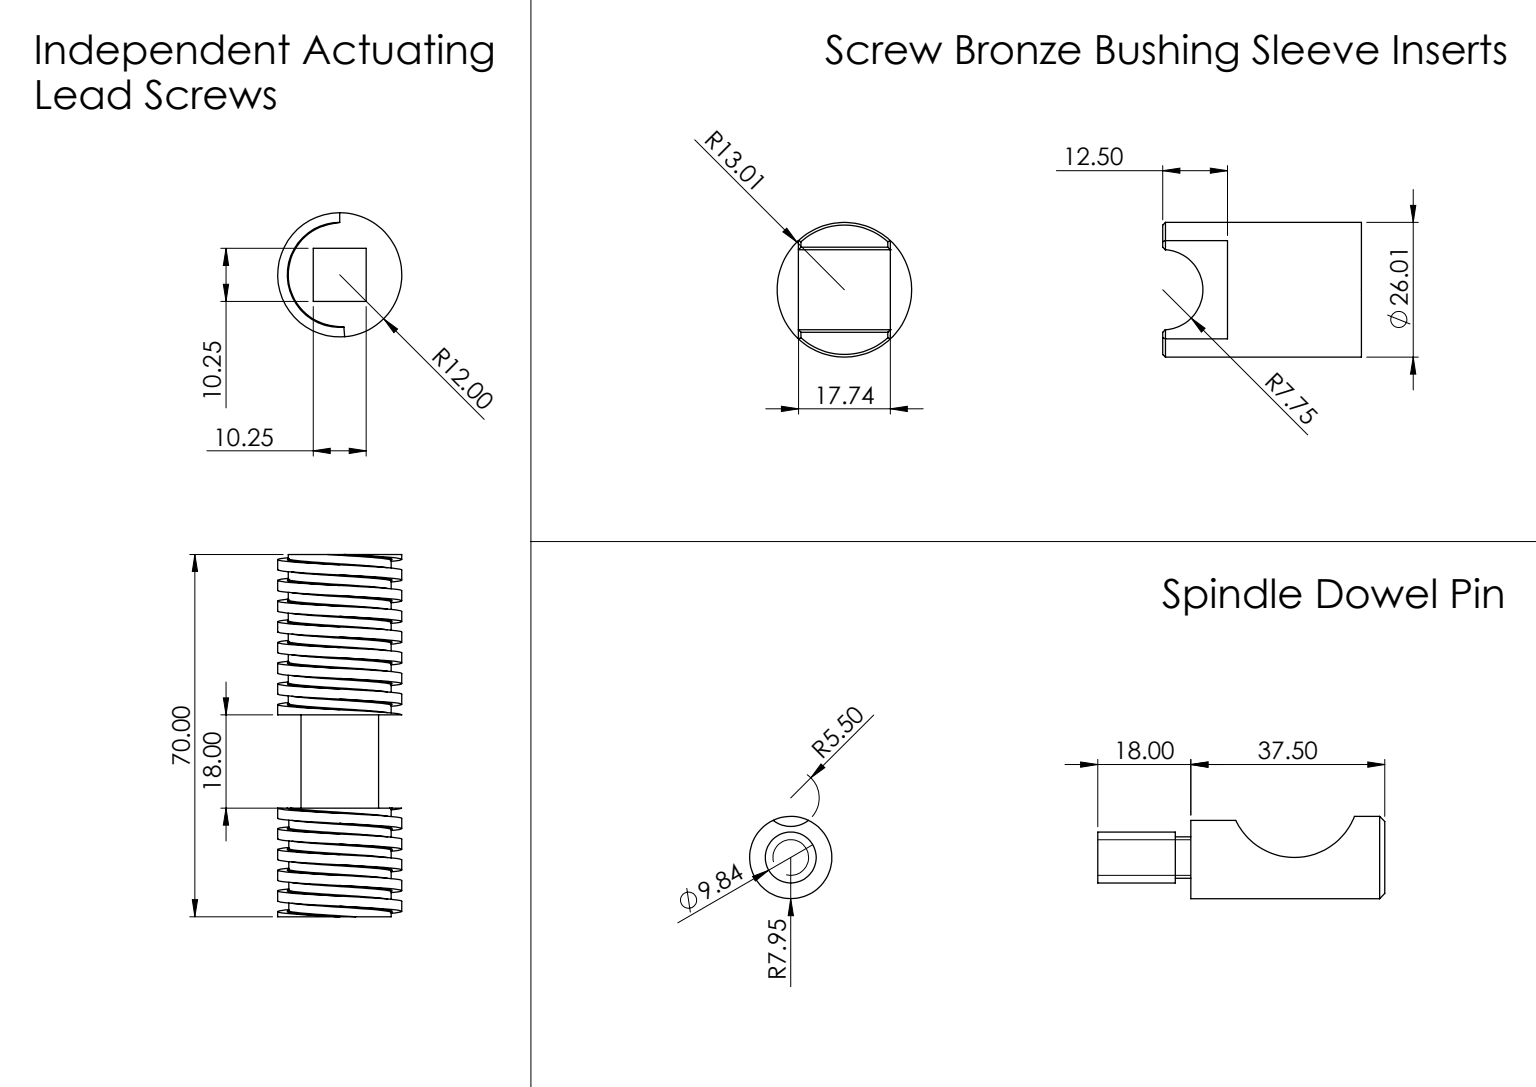
ISO-10303-21;
HEADER;
FILE_DESCRIPTION (('STEP AP214'),
    '1' );
FILE_NAME ('Spindle Dowel Pin.step',
    '2026-10-09T08:48:44',
    ( '' ),
    ( '' ),
    'SwSTEP 2.0',
    'SolidWorks 2026',
    '' );
FILE_SCHEMA (( 'AUTOMOTIVE_DESIGN' ));
ENDSEC;

DATA;
#25=CARTESIAN_POINT ( 'NONE',  ( 2.372150492836604986E-17, 0.000000000000000000, 0.1937007874015747588 ) ) ;
#117=CARTESIAN_POINT ( 'NONE',  ( 0.3074112942705509166, 1.261823755618582510, 0.05913325304464405602 ) ) ;
#225=DIRECTION ( 'NONE',  ( -0.000000000000000000, -1.000000000000000000, -0.000000000000000000 ) ) ;
#301=CARTESIAN_POINT ( 'NONE',  ( 0.000000000000000000, 2.185039370078740273, -0.2736220472440938911 ) ) ;
#383=EDGE_LOOP ( 'NONE', ( #46578, #71434, #76162, #29656 ) ) ;
#409=CARTESIAN_POINT ( 'NONE',  ( 0.01224130022169934474, 1.075705580628688152, 0.2362204724409448231 ) ) ;
#791=DIRECTION ( 'NONE',  ( 0.000000000000000000, 0.000000000000000000, -1.000000000000000000 ) ) ;
#799=DIRECTION ( 'NONE',  ( -0.000000000000000000, -1.000000000000000000, -0.000000000000000000 ) ) ;
#881=AXIS2_PLACEMENT_3D ( 'NONE', #25875, #225, #37687 ) ;
#969=CARTESIAN_POINT ( 'NONE',  ( 0.1341536278048623965, 1.050682278017460725, 0.2827841492639507348 ) ) ;
#1007=CARTESIAN_POINT ( 'NONE',  ( -0.2937696495028822574, 1.187747051217076910, 0.1083477314895111149 ) ) ;
#1152=CARTESIAN_POINT ( 'NONE',  ( 3.591975847892823865E-17, 2.185039370078740273, 0.2736220472440938911 ) ) ;
#1213=ORIENTED_EDGE ( 'NONE', *, *, #76419, .T. ) ;
#1243=VERTEX_POINT ( 'NONE', #14615 ) ;
#1297=ADVANCED_FACE ( 'NONE', ( #26383 ), #52458, .F. ) ;
#1417=CARTESIAN_POINT ( 'NONE',  ( -0.3126853129631109174, 1.368901411070787777, 0.01600703956764241986 ) ) ;
#1453=VERTEX_POINT ( 'NONE', #31866 ) ;
#1534=EDGE_LOOP ( 'NONE', ( #3579, #29369, #48090, #58856 ) ) ;
#2325=STYLED_ITEM ( 'NONE', ( #31329 ), #59000 ) ;
#2374=CARTESIAN_POINT ( 'NONE',  ( 0.3129921259842520787, 1.496062992125984259, 0.000000000000000000 ) ) ;
#2406=DIRECTION ( 'NONE',  ( 0.000000000000000000, 0.000000000000000000, 1.000000000000000000 ) ) ;
#2559=DIRECTION ( 'NONE',  ( 0.000000000000000000, 0.000000000000000000, -1.000000000000000000 ) ) ;
#2625=DIRECTION ( 'NONE',  ( 0.000000000000000000, 1.000000000000000000, 0.000000000000000000 ) ) ;
#2725=CARTESIAN_POINT ( 'NONE',  ( 3.833048050305355326E-17, 1.954428616053095924, 0.3129921259842520787 ) ) ;
#3026=DIRECTION ( 'NONE',  ( 0.000000000000000000, 0.000000000000000000, -1.000000000000000000 ) ) ;
#3140=CARTESIAN_POINT ( 'NONE',  ( 0.3126275856726307700, 1.620602844568471479, 0.01575678725321194573 ) ) ;
#3352=EDGE_CURVE ( 'NONE', #25849, #81942, #50111, .T. ) ;
#3373=VECTOR ( 'NONE', #51517, 39.37007874015748143 ) ;
#3384=FACE_OUTER_BOUND ( 'NONE', #39495, .T. ) ;
#3447=FACE_OUTER_BOUND ( 'NONE', #52967, .T. ) ;
#3556=CARTESIAN_POINT ( 'NONE',  ( 0.07836124490824399047, 1.950604500417927323, 0.3034306265812344305 ) ) ;
#3579=ORIENTED_EDGE ( 'NONE', *, *, #3352, .F. ) ;
#3625=LINE ( 'NONE', #47809, #52958 ) ;
#3671=CYLINDRICAL_SURFACE ( 'NONE', #57254, 0.3129921259842520787 ) ;
#3939=VERTEX_POINT ( 'NONE', #23651 ) ;
#3967=CARTESIAN_POINT ( 'NONE',  ( 0.2909691264735233540, 1.813546053633808830, 0.1157836905918017273 ) ) ;
#4054=CARTESIAN_POINT ( 'NONE',  ( -0.1341536278048670039, 1.050682278017461835, 0.2827841492639485144 ) ) ;
#4079=DIRECTION ( 'NONE',  ( -0.000000000000000000, -1.000000000000000000, -0.000000000000000000 ) ) ;
#4201=CARTESIAN_POINT ( 'NONE',  ( 0.000000000000000000, 2.145669291338582418, -0.3129921259842520787 ) ) ;
#4609=DIRECTION ( 'NONE',  ( 0.000000000000000000, 0.000000000000000000, -1.000000000000000000 ) ) ;
#5256=SURFACE_SIDE_STYLE ('',( #44356 ) ) ;
#5276=CARTESIAN_POINT ( 'NONE',  ( -0.1224964469087656410, 1.944119274041657519, 0.2884380004297487088 ) ) ;
#5295=ORIENTED_EDGE ( 'NONE', *, *, #11474, .F. ) ;
#5671=ORIENTED_EDGE ( 'NONE', *, *, #32566, .T. ) ;
#5679=CARTESIAN_POINT ( 'NONE',  ( 3.833048050305355326E-17, 1.954428616053095924, 0.3129921259842520787 ) ) ;
#5999=AXIS2_PLACEMENT_3D ( 'NONE', #65318, #14396, #38786 ) ;
#6197=ORIENTED_EDGE ( 'NONE', *, *, #68902, .T. ) ;
#6325=AXIS2_PLACEMENT_3D ( 'NONE', #24341, #42454, #56734 ) ;
#6346=ADVANCED_FACE ( 'NONE', ( #36689, #61550 ), #81335, .T. ) ;
#6925=LINE ( 'NONE', #78486, #3373 ) ;
#7227=ORIENTED_EDGE ( 'NONE', *, *, #28583, .T. ) ;
#7263=CARTESIAN_POINT ( 'NONE',  ( 0.3104096989839266740, 1.295945406154406454, 0.04180176832660051356 ) ) ;
#7469=DIRECTION ( 'NONE',  ( -0.000000000000000000, -1.000000000000000000, -0.000000000000000000 ) ) ;
#7519=VERTEX_POINT ( 'NONE', #4201 ) ;
#7675=VECTOR ( 'NONE', #22908, 39.37007874015748143 ) ;
#7733=CARTESIAN_POINT ( 'NONE',  ( -0.3129921259842520231, 1.470107679032609971, 3.734948428837856094E-17 ) ) ;
#7767=CARTESIAN_POINT ( 'NONE',  ( 0.000000000000000000, 0.000000000000000000, 0.000000000000000000 ) ) ;
#7885=ORIENTED_EDGE ( 'NONE', *, *, #20353, .F. ) ;
#7890=CARTESIAN_POINT ( 'NONE',  ( -0.04868480690927201593, 1.072582076400621753, 0.2414116071904397476 ) ) ;
#7943=ADVANCED_FACE ( 'NONE', ( #3384 ), #56554, .T. ) ;
#8076=ORIENTED_EDGE ( 'NONE', *, *, #32566, .F. ) ;
#8107=CARTESIAN_POINT ( 'NONE',  ( 0.2748794045270251951, 1.142111962221293409, 0.1499919135227574252 ) ) ;
#8145=CARTESIAN_POINT ( 'NONE',  ( -0.2835710216259798577, 1.159555538018685716, 0.1328243903749163624 ) ) ;
#8310=DIRECTION ( 'NONE',  ( 1.000000000000000000, -0.000000000000000000, -0.000000000000000000 ) ) ;
#8366=PRODUCT ( 'Spindle Dowel Pin', 'Spindle Dowel Pin', '', ( #30024 ) ) ;
#8391=CARTESIAN_POINT ( 'NONE',  ( 0.1341536278048623965, 1.050682278017460725, 0.2827841492639507348 ) ) ;
#8564=ORIENTED_EDGE ( 'NONE', *, *, #32130, .F. ) ;
#8617=VERTEX_POINT ( 'NONE', #32503 ) ;
#8933=PLANE ( 'NONE',  #11755 ) ;
#8939=CIRCLE ( 'NONE', #74851, 0.1937007874015748143 ) ;
#8988=EDGE_CURVE ( 'NONE', #3939, #18816, #67404, .T. ) ;
#9096=EDGE_LOOP ( 'NONE', ( #28412, #46874, #14400, #76473, #66041, #66129, #8076 ) ) ;
#9136=CARTESIAN_POINT ( 'NONE',  ( 0.000000000000000000, 0.000000000000000000, 0.000000000000000000 ) ) ;
#9758=AXIS2_PLACEMENT_3D ( 'NONE', #68690, #23649, #53976 ) ;
#9868=CARTESIAN_POINT ( 'NONE',  ( 0.3130345246323552599, 1.559122693537392745, 0.003049358274158167365 ) ) ;
#10309=ADVANCED_FACE ( 'NONE', ( #27240 ), #73542, .F. ) ;
#10351=SURFACE_STYLE_USAGE ( .BOTH. , #5256 ) ;
#10361=EDGE_LOOP ( 'NONE', ( #73166, #30222 ) ) ;
#10364=DIRECTION ( 'NONE',  ( 0.000000000000000000, 0.000000000000000000, -1.000000000000000000 ) ) ;
#10589=DIRECTION ( 'NONE',  ( 0.000000000000000000, -1.000000000000000000, 0.000000000000000000 ) ) ;
#10777=CARTESIAN_POINT ( 'NONE',  ( -0.3072632741606444173, 1.737537999042348513, 0.06216925787398272507 ) ) ;
#11014=ADVANCED_FACE ( 'NONE', ( #38097 ), #76103, .T. ) ;
#11188=CARTESIAN_POINT ( 'NONE',  ( 0.000000000000000000, 0.5905511811023621549, -0.1937007874015747588 ) ) ;
#11190=CARTESIAN_POINT ( 'NONE',  ( -0.2493074132419488831, 1.884549279140503408, 0.1897364805620621597 ) ) ;
#11276=ORIENTED_EDGE ( 'NONE', *, *, #37551, .F. ) ;
#11474=EDGE_CURVE ( 'NONE', #16433, #18816, #43794, .T. ) ;
#11755=AXIS2_PLACEMENT_3D ( 'NONE', #72906, #2625, #79656 ) ;
#11869=CIRCLE ( 'NONE', #50650, 0.3129921259842521897 ) ;
#12372=ADVANCED_FACE ( 'NONE', ( #28796 ), #80173, .F. ) ;
#12411=EDGE_LOOP ( 'NONE', ( #77639, #27414 ) ) ;
#12421=CARTESIAN_POINT ( 'NONE',  ( -0.1887375355206090954, 1.924695534443318090, 0.2501427588384230183 ) ) ;
#12546=AXIS2_PLACEMENT_3D ( 'NONE', #74485, #47545, #54688 ) ;
#12711=EDGE_LOOP ( 'NONE', ( #79365, #14090, #71316, #31641, #37257 ) ) ;
#13043=CARTESIAN_POINT ( 'NONE',  ( 0.02439311036560904908, 1.075073066373593234, 0.2372510453448407330 ) ) ;
#13195=CARTESIAN_POINT ( 'NONE',  ( 0.1341536278048623410, 0.7086614173228346081, 0.2827841492639508458 ) ) ;
#13216=CARTESIAN_POINT ( 'NONE',  ( -0.3130110660353679908, 1.444485302887537514, 0.002040369744756952066 ) ) ;
#13353=CARTESIAN_POINT ( 'NONE',  ( 0.000000000000000000, 0.5905511811023621549, 0.000000000000000000 ) ) ;
#13876=DIRECTION ( 'NONE',  ( 0.000000000000000000, -0.7071067811865437980, -0.7071067811865511255 ) ) ;
#14020=CIRCLE ( 'NONE', #24744, 0.1574803149606299746 ) ;
#14090=ORIENTED_EDGE ( 'NONE', *, *, #52104, .T. ) ;
#14206=VERTEX_POINT ( 'NONE', #68041 ) ;
#14207=EDGE_LOOP ( 'NONE', ( #60952, #75599, #55224, #46243, #18435, #5295, #68335 ) ) ;
#14304=CARTESIAN_POINT ( 'NONE',  ( -2.199130528046420221E-22, 1.075705580628688596, 0.2362204724409449064 ) ) ;
#14378=VERTEX_POINT ( 'NONE', #4054 ) ;
#14396=DIRECTION ( 'NONE',  ( 1.000000000000000000, -0.000000000000000000, -0.000000000000000000 ) ) ;
#14400=ORIENTED_EDGE ( 'NONE', *, *, #56918, .T. ) ;
#14472=CARTESIAN_POINT ( 'NONE',  ( -0.3064070226227782467, 1.250422264350145474, 0.06492945659560576954 ) ) ;
#14549=EDGE_CURVE ( 'NONE', #39843, #58335, #44637, .T. ) ;
#14607=DIRECTION ( 'NONE',  ( -0.000000000000000000, -1.000000000000000000, -0.000000000000000000 ) ) ;
#14615=CARTESIAN_POINT ( 'NONE',  ( 3.833048052449394218E-17, 2.145669291338582418, 0.3129921259842520787 ) ) ;
#14719=CARTESIAN_POINT ( 'NONE',  ( 0.09404056145105300912, 1.063503333403748474, 0.2573448916946036724 ) ) ;
#14869=ADVANCED_FACE ( 'NONE', ( #3447 ), #8933, .T. ) ;
#15024=LINE ( 'NONE', #40680, #28369 ) ;
#15036=CARTESIAN_POINT ( 'NONE',  ( -0.06038700950485487162, 1.070773487107445909, 0.2444607762650621019 ) ) ;
#15218=VERTEX_POINT ( 'NONE', #71137 ) ;
#15385=EDGE_LOOP ( 'NONE', ( #22971, #11276 ) ) ;
#15414=VERTEX_POINT ( 'NONE', #64400 ) ;
#15463=DIRECTION ( 'NONE',  ( 0.000000000000000000, 0.000000000000000000, -1.000000000000000000 ) ) ;
#15486=CARTESIAN_POINT ( 'NONE',  ( 0.000000000000000000, -1.268531780058464091E-17, 0.000000000000000000 ) ) ;
#15994=B_SPLINE_CURVE_WITH_KNOTS ( 'NONE', 3,
 ( #8391, #26493, #78693, #14719, #77427, #52563, #51725, #13043, #409, #14304 ),
 .UNSPECIFIED., .F., .F.,
 ( 4, 2, 2, 2, 4 ),
 ( 0.001464733143057391418, 0.002397049282983275756, 0.003329365422909159877, 0.004261681562835043131, 0.005193997702760927253 ),
 .UNSPECIFIED. ) ;
#16286=SHAPE_REPRESENTATION_RELATIONSHIP ( 'NONE' , 'NONE' ,  #76132, #64521 ) ;
#16312=DIRECTION ( 'NONE',  ( 0.000000000000000000, 0.000000000000000000, -1.000000000000000000 ) ) ;
#16433=VERTEX_POINT ( 'NONE', #55908 ) ;
#16485=EDGE_CURVE ( 'NONE', #1243, #7519, #53371, .T. ) ;
#16560=CARTESIAN_POINT ( 'NONE',  ( -0.1341536278048623410, 0.7086614173228346081, 0.2827841492639507903 ) ) ;
#16609=CARTESIAN_POINT ( 'NONE',  ( 0.2009426810023753340, 1.919101783098011715, 0.2404105009256824188 ) ) ;
#16873=DIRECTION ( 'NONE',  ( -0.000000000000000000, -1.000000000000000000, -0.000000000000000000 ) ) ;
#17028=CARTESIAN_POINT ( 'NONE',  ( 0.2320225394537987207, 1.899862155193571711, 0.2105147107788077343 ) ) ;
#17085=FILL_AREA_STYLE ('',( #74737 ) ) ;
#17106=CARTESIAN_POINT ( 'NONE',  ( -0.2867050620510094849, 1.825346416092846091, 0.1260848743807634342 ) ) ;
#17210=PLANE ( 'NONE',  #57386 ) ;
#17274=DIRECTION ( 'NONE',  ( -0.000000000000000000, -1.000000000000000000, -0.000000000000000000 ) ) ;
#17515=CARTESIAN_POINT ( 'NONE',  ( -0.2570577095524356759, 1.875999552332453746, 0.1790154821377908934 ) ) ;
#17897=EDGE_CURVE ( 'NONE', #75063, #3939, #42675, .T. ) ;
#17903=( NAMED_UNIT ( * ) SI_UNIT ( $, .STERADIAN. ) SOLID_ANGLE_UNIT ( ) );
#17914=ORIENTED_EDGE ( 'NONE', *, *, #3352, .T. ) ;
#17922=CARTESIAN_POINT ( 'NONE',  ( -0.3129921259842520787, 1.496062992125984259, 2.300774849103979725E-17 ) ) ;
#18007=ORIENTED_EDGE ( 'NONE', *, *, #11474, .T. ) ;
#18252=CARTESIAN_POINT ( 'NONE',  ( 0.000000000000000000, 0.000000000000000000, 0.000000000000000000 ) ) ;
#18429=DIRECTION ( 'NONE',  ( 0.000000000000000000, 0.000000000000000000, -1.000000000000000000 ) ) ;
#18435=ORIENTED_EDGE ( 'NONE', *, *, #32130, .T. ) ;
#18636=DIRECTION ( 'NONE',  ( 0.000000000000000000, 1.000000000000000000, 0.000000000000000000 ) ) ;
#18816=VERTEX_POINT ( 'NONE', #13195 ) ;
#19735=ORIENTED_EDGE ( 'NONE', *, *, #20396, .F. ) ;
#19797=AXIS2_PLACEMENT_3D ( 'NONE', #23157, #16873, #61876 ) ;
#19980=EDGE_CURVE ( 'NONE', #39843, #75063, #15994, .T. ) ;
#20353=EDGE_CURVE ( 'NONE', #49008, #14378, #70690, .T. ) ;
#20385=DIRECTION ( 'NONE',  ( 0.000000000000000000, 0.000000000000000000, -1.000000000000000000 ) ) ;
#20396=EDGE_CURVE ( 'NONE', #31638, #7519, #45830, .T. ) ;
#20602=CARTESIAN_POINT ( 'NONE',  ( 0.000000000000000000, 0.000000000000000000, 0.000000000000000000 ) ) ;
#20680=ORIENTED_EDGE ( 'NONE', *, *, #53659, .T. ) ;
#20733=CARTESIAN_POINT ( 'NONE',  ( 0.2527386706991758825, 1.111414106920971090, 0.1849575905693944811 ) ) ;
#20828=DIRECTION ( 'NONE',  ( 0.000000000000000000, 0.000000000000000000, -1.000000000000000000 ) ) ;
#21132=COLOUR_RGB ( '', 0.08235294, 0.09019608, 0.10196078) ;
#21148=CARTESIAN_POINT ( 'NONE',  ( 0.3114547874990893916, 1.319604222443112151, 0.03199850469859417956 ) ) ;
#21435=VERTEX_POINT ( 'NONE', #11188 ) ;
#21647=DIRECTION ( 'NONE',  ( 0.000000000000000000, 0.000000000000000000, -1.000000000000000000 ) ) ;
#21660=CARTESIAN_POINT ( 'NONE',  ( 0.2979138814448422101, 1.789193252437325743, 0.09652054087235428792 ) ) ;
#21737=DIRECTION ( 'NONE',  ( -0.000000000000000000, -1.000000000000000000, -0.000000000000000000 ) ) ;
#21748=CARTESIAN_POINT ( 'NONE',  ( -0.02462164107398554652, 1.075056246094946211, 0.2372787660107268937 ) ) ;
#21844=CARTESIAN_POINT ( 'NONE',  ( 0.1341536278048623965, 1.050682278017460725, 0.2827841492639507348 ) ) ;
#22077=CARTESIAN_POINT ( 'NONE',  ( 0.1230917936933036416, 1.944006284485450209, 0.2881873359806741419 ) ) ;
#22098=AXIS2_PLACEMENT_3D ( 'NONE', #9136, #2406, #28064 ) ;
#22901=CARTESIAN_POINT ( 'NONE',  ( 0.3095674345919382509, 1.709700804348449843, 0.04767548262574627937 ) ) ;
#22908=DIRECTION ( 'NONE',  ( -0.000000000000000000, -1.000000000000000000, -0.000000000000000000 ) ) ;
#22971=ORIENTED_EDGE ( 'NONE', *, *, #57708, .F. ) ;
#23157=CARTESIAN_POINT ( 'NONE',  ( 0.000000000000000000, 0.000000000000000000, 0.000000000000000000 ) ) ;
#23169=ORIENTED_EDGE ( 'NONE', *, *, #28151, .T. ) ;
#23314=CARTESIAN_POINT ( 'NONE',  ( 0.2451238321738833381, 1.888229281464673948, 0.1947436408813261743 ) ) ;
#23327=DIRECTION ( 'NONE',  ( 8.659560562354975999E-17, -0.7071067811865437980, 0.7071067811865511255 ) ) ;
#23385=FACE_OUTER_BOUND ( 'NONE', #1534, .T. ) ;
#23649=DIRECTION ( 'NONE',  ( 0.000000000000000000, -1.000000000000000000, -0.000000000000000000 ) ) ;
#23651=CARTESIAN_POINT ( 'NONE',  ( 0.000000000000000000, 0.7086614173228346081, 0.2362204724409449064 ) ) ;
#23816=( CONVERSION_BASED_UNIT ( 'INCH', #36040 ) LENGTH_UNIT ( ) NAMED_UNIT ( #43771 ) );
#23849=CARTESIAN_POINT ( 'NONE',  ( 1.928577636452524918E-17, 0.000000000000000000, 0.1574803149606299746 ) ) ;
#24212=CARTESIAN_POINT ( 'NONE',  ( -0.3130349471939997685, 1.559138852304699174, 0.003046472099445048272 ) ) ;
#24317=CARTESIAN_POINT ( 'NONE',  ( 0.1937007874015748143, -6.342658900292320455E-18, 0.000000000000000000 ) ) ;
#24339=AXIS2_PLACEMENT_3D ( 'NONE', #76558, #32762, #791 ) ;
#24341=CARTESIAN_POINT ( 'NONE',  ( 0.000000000000000000, 2.145669291338582418, 0.000000000000000000 ) ) ;
#24430=DIMENSIONAL_EXPONENTS ( 1.000000000000000000, 0.000000000000000000, 0.000000000000000000, 0.000000000000000000, 0.000000000000000000, 0.000000000000000000, 0.000000000000000000 ) ;
#24744=AXIS2_PLACEMENT_3D ( 'NONE', #44138, #17274, #4609 ) ;
#25004=AXIS2_PLACEMENT_3D ( 'NONE', #18252, #31274, #56939 ) ;
#25084=EDGE_CURVE ( 'NONE', #69331, #81942, #62659, .T. ) ;
#25849=VERTEX_POINT ( 'NONE', #81088 ) ;
#25875=CARTESIAN_POINT ( 'NONE',  ( 0.000000000000000000, 2.145669291338582418, 0.000000000000000000 ) ) ;
#25958=DIRECTION ( 'NONE',  ( -0.000000000000000000, -1.000000000000000000, -0.000000000000000000 ) ) ;
#26140=ORIENTED_EDGE ( 'NONE', *, *, #37551, .T. ) ;
#26383=FACE_OUTER_BOUND ( 'NONE', #33205, .T. ) ;
#26401=AXIS2_PLACEMENT_3D ( 'NONE', #40701, #8310, #15463 ) ;
#26492=CYLINDRICAL_SURFACE ( 'NONE', #73490, 0.1937007874015747588 ) ;
#26493=CARTESIAN_POINT ( 'NONE',  ( 0.1249024489578631214, 1.054114278624317835, 0.2754824702603712039 ) ) ;
#26623=CARTESIAN_POINT ( 'NONE',  ( 0.1876687465225647666, 1.067092265285233266, 0.2507773264951494996 ) ) ;
#26693=CYLINDRICAL_SURFACE ( 'NONE', #77547, 0.1574803149606299746 ) ;
#26815=CARTESIAN_POINT ( 'NONE',  ( -0.08317555404016972742, 1.066210426301412717, 0.2524679153701900325 ) ) ;
#27002=ADVANCED_FACE ( 'NONE', ( #66053 ), #26492, .T. ) ;
#27032=CARTESIAN_POINT ( 'NONE',  ( 0.3129921259842522452, 1.470238543415450350, 1.333910153156375395E-19 ) ) ;
#27056=DIRECTION ( 'NONE',  ( 0.000000000000000000, 0.000000000000000000, -1.000000000000000000 ) ) ;
#27240=FACE_OUTER_BOUND ( 'NONE', #12711, .T. ) ;
#27414=ORIENTED_EDGE ( 'NONE', *, *, #49189, .F. ) ;
#27449=CARTESIAN_POINT ( 'NONE',  ( 0.3011055150036106021, 1.218137231435314272, 0.08579257120109930190 ) ) ;
#27907=CARTESIAN_POINT ( 'NONE',  ( -0.3104009647183427756, 1.295819047631763254, 0.04186094777090585556 ) ) ;
#28064=DIRECTION ( 'NONE',  ( 1.000000000000000000, 0.000000000000000000, 0.000000000000000000 ) ) ;
#28151=EDGE_CURVE ( 'NONE', #21435, #25849, #45776, .T. ) ;
#28319=CARTESIAN_POINT ( 'NONE',  ( -0.1341536278048670039, 1.050682278017461835, 0.2827841492639485144 ) ) ;
#28369=VECTOR ( 'NONE', #21737, 39.37007874015748143 ) ;
#28412=ORIENTED_EDGE ( 'NONE', *, *, #36496, .F. ) ;
#28496=UNCERTAINTY_MEASURE_WITH_UNIT (LENGTH_MEASURE( 1.000000000000000082E-05 ), #81468, 'distance_accuracy_value', 'NONE');
#28541=VERTEX_POINT ( 'NONE', #1152 ) ;
#28583=EDGE_CURVE ( 'NONE', #1453, #8617, #30996, .T. ) ;
#28796=FACE_OUTER_BOUND ( 'NONE', #68835, .T. ) ;
#28803=CARTESIAN_POINT ( 'NONE',  ( 0.2570685524539542688, 1.875513320822418839, 0.1786727789893264307 ) ) ;
#28886=PRODUCT_DEFINITION_FORMATION_WITH_SPECIFIED_SOURCE ( 'ANY', '', #8366, .NOT_KNOWN. ) ;
#28893=FACE_OUTER_BOUND ( 'NONE', #12411, .T. ) ;
#29148=CARTESIAN_POINT ( 'NONE',  ( -0.2589415859896363470, 1.118607810292596705, 0.1761306047597130386 ) ) ;
#29369=ORIENTED_EDGE ( 'NONE', *, *, #49189, .T. ) ;
#29615=SHAPE_DEFINITION_REPRESENTATION ( #60807, #76132 ) ;
#29630=CARTESIAN_POINT ( 'NONE',  ( 0.1083363854164813983, 1.946602136093918745, 0.2940643763633090102 ) ) ;
#29656=ORIENTED_EDGE ( 'NONE', *, *, #53659, .F. ) ;
#30024=PRODUCT_CONTEXT ( 'NONE', #61604, 'mechanical' ) ;
#30068=EDGE_CURVE ( 'NONE', #49008, #3939, #66058, .T. ) ;
#30099=( LENGTH_UNIT ( ) NAMED_UNIT ( * ) SI_UNIT ( $, .METRE. ) );
#30118=CARTESIAN_POINT ( 'NONE',  ( -0.06257671775081299903, 1.952079521258549777, 0.3070762858441002940 ) ) ;
#30222=ORIENTED_EDGE ( 'NONE', *, *, #73238, .T. ) ;
#30517=( NAMED_UNIT ( * ) PLANE_ANGLE_UNIT ( ) SI_UNIT ( $, .RADIAN. ) );
#30555=EDGE_LOOP ( 'NONE', ( #23169, #17914, #39523, #35275 ) ) ;
#30641=FACE_OUTER_BOUND ( 'NONE', #10361, .T. ) ;
#30939=CARTESIAN_POINT ( 'NONE',  ( -0.1637150164629772586, 1.933882213591592736, 0.2671902889294776595 ) ) ;
#30996=CIRCLE ( 'NONE', #80787, 0.1574803149606299746 ) ;
#31274=DIRECTION ( 'NONE',  ( -0.000000000000000000, -1.000000000000000000, -0.000000000000000000 ) ) ;
#31329=PRESENTATION_STYLE_ASSIGNMENT (( #10351 ) ) ;
#31638=VERTEX_POINT ( 'NONE', #301 ) ;
#31641=ORIENTED_EDGE ( 'NONE', *, *, #19980, .F. ) ;
#31866=CARTESIAN_POINT ( 'NONE',  ( 0.000000000000000000, 0.5905511811023621549, -0.1574803149606299746 ) ) ;
#32108=PRODUCT_DEFINITION ( 'UNKNOWN', '', #28886, #61306 ) ;
#32130=EDGE_CURVE ( 'NONE', #39843, #18816, #15024, .T. ) ;
#32293=DIRECTION ( 'NONE',  ( 0.000000000000000000, 0.000000000000000000, -1.000000000000000000 ) ) ;
#32503=CARTESIAN_POINT ( 'NONE',  ( 1.928577636452524918E-17, 0.5905511811023621549, 0.1574803149606299746 ) ) ;
#32511=CARTESIAN_POINT ( 'NONE',  ( 0.2063662664111909073, 1.075973491904217871, 0.2356306219338031305 ) ) ;
#32566=EDGE_CURVE ( 'NONE', #14206, #15218, #40961, .T. ) ;
#32698=DIRECTION ( 'NONE',  ( -0.000000000000000000, -1.000000000000000000, -0.000000000000000000 ) ) ;
#32762=DIRECTION ( 'NONE',  ( 0.000000000000000000, -1.000000000000000000, 0.000000000000000000 ) ) ;
#32895=FACE_OUTER_BOUND ( 'NONE', #54214, .T. ) ;
#32971=CARTESIAN_POINT ( 'NONE',  ( -0.3129921259842520787, 1.496062992125984259, 2.300774849103979725E-17 ) ) ;
#33200=( GEOMETRIC_REPRESENTATION_CONTEXT ( 3 ) GLOBAL_UNCERTAINTY_ASSIGNED_CONTEXT ( ( #28496 ) ) GLOBAL_UNIT_ASSIGNED_CONTEXT ( ( #81468, #30517, #17903 ) ) REPRESENTATION_CONTEXT ( 'NONE', 'WORKASPACE' ) );
#33205=EDGE_LOOP ( 'NONE', ( #48733, #76091, #39632, #8564 ) ) ;
#33330=ORIENTED_EDGE ( 'NONE', *, *, #43286, .T. ) ;
#33362=CARTESIAN_POINT ( 'NONE',  ( 0.2314737228097724919, 1.092014648053644565, 0.2109979669470876118 ) ) ;
#33400=CARTESIAN_POINT ( 'NONE',  ( -0.3128565372736722416, 1.393882159635214890, 0.01004378685656346325 ) ) ;
#33733=EDGE_CURVE ( 'NONE', #31638, #28541, #36477, .T. ) ;
#33773=CARTESIAN_POINT ( 'NONE',  ( 0.3130111271098954262, 1.444537301488023839, 0.002033853763896861528 ) ) ;
#33784=DIRECTION ( 'NONE',  ( -0.000000000000000000, -1.000000000000000000, -0.000000000000000000 ) ) ;
#34267=ORIENTED_EDGE ( 'NONE', *, *, #30068, .T. ) ;
#34422=B_SPLINE_CURVE_WITH_KNOTS ( 'NONE', 3,
 ( #78181, #45743, #21748, #7890, #15036, #26815, #39443, #72688, #46995, #53721 ),
 .UNSPECIFIED., .F., .F.,
 ( 4, 2, 2, 2, 4 ),
 ( 0.005193997702760927253, 0.006123015815168760499, 0.007052033927576592878, 0.007981052039984426125, 0.008910070152392259371 ),
 .UNSPECIFIED. ) ;
#34543=CARTESIAN_POINT ( 'NONE',  ( 0.000000000000000000, 2.145669291338582418, 0.000000000000000000 ) ) ;
#34588=VECTOR ( 'NONE', #37121, 39.37007874015748143 ) ;
#34716=CARTESIAN_POINT ( 'NONE',  ( 0.3129921259842522452, 1.527841585044882100, -3.001297844601851921E-19 ) ) ;
#34834=DIRECTION ( 'NONE',  ( -0.000000000000000000, -1.000000000000000000, -0.000000000000000000 ) ) ;
#35275=ORIENTED_EDGE ( 'NONE', *, *, #79779, .F. ) ;
#35369=DIRECTION ( 'NONE',  ( -0.000000000000000000, -1.000000000000000000, -0.000000000000000000 ) ) ;
#35498=VECTOR ( 'NONE', #4079, 39.37007874015748143 ) ;
#35512=DIRECTION ( 'NONE',  ( 0.000000000000000000, 0.000000000000000000, -1.000000000000000000 ) ) ;
#35515=CIRCLE ( 'NONE', #73132, 0.3129921259842520787 ) ;
#35537=CARTESIAN_POINT ( 'NONE',  ( 0.2868249070713367876, 1.825030329442032917, 0.1258042619966805165 ) ) ;
#35564=EDGE_CURVE ( 'NONE', #58335, #14206, #68976, .T. ) ;
#35627=( LENGTH_UNIT ( ) NAMED_UNIT ( * ) SI_UNIT ( $, .METRE. ) );
#35720=DIRECTION ( 'NONE',  ( 0.000000000000000000, 0.000000000000000000, 1.000000000000000000 ) ) ;
#35884=CARTESIAN_POINT ( 'NONE',  ( -0.1775461242611900137, 1.063099670987233569, 0.2580608039878784510 ) ) ;
#35963=CARTESIAN_POINT ( 'NONE',  ( 0.000000000000000000, 2.185078740157480937, 0.2362204724409449064 ) ) ;
#36040=LENGTH_MEASURE_WITH_UNIT ( LENGTH_MEASURE( 0.02539999999999999897 ), #35627 );
#36127=ORIENTED_EDGE ( 'NONE', *, *, #65474, .T. ) ;
#36288=CARTESIAN_POINT ( 'NONE',  ( -0.2526890999533557003, 1.111360978596734883, 0.1850246388144368703 ) ) ;
#36321=ADVANCED_FACE ( 'NONE', ( #49806 ), #49398, .T. ) ;
#36477=CIRCLE ( 'NONE', #62017, 0.2736220472440938911 ) ;
#36496=EDGE_CURVE ( 'NONE', #1243, #14206, #64935, .T. ) ;
#36689=FACE_OUTER_BOUND ( 'NONE', #65322, .T. ) ;
#36704=LINE ( 'NONE', #62378, #34588 ) ;
#36831=LENGTH_MEASURE_WITH_UNIT ( LENGTH_MEASURE( 0.02539999999999999897 ), #30099 );
#37121=DIRECTION ( 'NONE',  ( 1.000000000000000000, -0.000000000000000000, -0.000000000000000000 ) ) ;
#37257=ORIENTED_EDGE ( 'NONE', *, *, #14549, .T. ) ;
#37260=CYLINDRICAL_SURFACE ( 'NONE', #69081, 0.1937007874015747588 ) ;
#37551=EDGE_CURVE ( 'NONE', #75751, #15414, #39876, .T. ) ;
#37666=CARTESIAN_POINT ( 'NONE',  ( -0.2217488924428978880, 1.907169838053261124, 0.2213636967189943072 ) ) ;
#37687=DIRECTION ( 'NONE',  ( 0.000000000000000000, 0.000000000000000000, -1.000000000000000000 ) ) ;
#38097=FACE_OUTER_BOUND ( 'NONE', #79100, .T. ) ;
#38247=CARTESIAN_POINT ( 'NONE',  ( 0.000000000000000000, 0.000000000000000000, -0.1574803149606299746 ) ) ;
#38252=VECTOR ( 'NONE', #799, 39.37007874015748143 ) ;
#38696=CARTESIAN_POINT ( 'NONE',  ( -0.1341536278048623410, 1.446850393700787274, 0.2827841492639507903 ) ) ;
#38786=DIRECTION ( 'NONE',  ( 0.000000000000000000, 0.000000000000000000, -1.000000000000000000 ) ) ;
#38862=CARTESIAN_POINT ( 'NONE',  ( -0.3034767870060118278, 1.228735513192457551, 0.07815720285223907993 ) ) ;
#39241=CARTESIAN_POINT ( 'NONE',  ( 0.1565873217565743603, 1.056201437308684321, 0.2712946218330505865 ) ) ;
#39443=CARTESIAN_POINT ( 'NONE',  ( -0.09423411257991823331, 1.063451938596666979, 0.2574397322871235794 ) ) ;
#39495=EDGE_LOOP ( 'NONE', ( #79987, #58306, #42841, #67716 ) ) ;
#39523=ORIENTED_EDGE ( 'NONE', *, *, #25084, .F. ) ;
#39632=ORIENTED_EDGE ( 'NONE', *, *, #8988, .T. ) ;
#39667=CARTESIAN_POINT ( 'NONE',  ( 0.1777261984983631582, 1.063163173673139505, 0.2579413877952805856 ) ) ;
#39843=VERTEX_POINT ( 'NONE', #21844 ) ;
#39876=CIRCLE ( 'NONE', #51918, 0.1574803149606299746 ) ;
#40126=CARTESIAN_POINT ( 'NONE',  ( -0.2872938682423638590, 1.168647385053847909, 0.1245073136739714287 ) ) ;
#40269=DIRECTION ( 'NONE',  ( 0.000000000000000000, 0.000000000000000000, -1.000000000000000000 ) ) ;
#40409=ADVANCED_FACE ( 'NONE', ( #30641 ), #17210, .T. ) ;
#40482=AXIS2_PLACEMENT_3D ( 'NONE', #34543, #35369, #2559 ) ;
#40680=CARTESIAN_POINT ( 'NONE',  ( 0.1341536278048623410, 1.446850393700787274, 0.2827841492639507903 ) ) ;
#40701=CARTESIAN_POINT ( 'NONE',  ( -0.3129921259842521897, 1.496062992125984259, 0.4921259842519685179 ) ) ;
#40780=DIRECTION ( 'NONE',  ( 0.000000000000000000, 0.000000000000000000, -1.000000000000000000 ) ) ;
#40961=B_SPLINE_CURVE_WITH_KNOTS ( 'NONE', 3,
 ( #5679, #44374, #69669, #30118, #74758, #82709, #5276, #56200, #30939, #12421, #56606, #37666, #57013, #11190, #17515, #63753, #57429, #17106, #43147, #68437, #55780, #10777, #62110, #81901, #81488, #24212, #75583, #17922 ),
 .UNSPECIFIED., .F., .F.,
 ( 4, 2, 2, 2, 2, 2, 2, 2, 2, 2, 2, 2, 2, 4 ),
 ( 0.01911876323414707021, 0.02031104709728144900, 0.02150333096041582431, 0.02269561482355020310, 0.02388789868668458188, 0.02508018254981896067, 0.02627246641295333945, 0.02746475027608771824, 0.02865703413922209702, 0.02984931800235647581, 0.03104160186549084766, 0.03342616959175960523, 0.03581073731802836280, 0.03819530504429712037 ),
 .UNSPECIFIED. ) ;
#40993=DIRECTION ( 'NONE',  ( -0.000000000000000000, -1.000000000000000000, -0.000000000000000000 ) ) ;
#41095=VECTOR ( 'NONE', #13876, 39.37007874015748854 ) ;
#41423=DIRECTION ( 'NONE',  ( -0.000000000000000000, -1.000000000000000000, -0.000000000000000000 ) ) ;
#41436=CARTESIAN_POINT ( 'NONE',  ( 0.1509182436465724975, 1.937587712771704940, 0.2746401537082780453 ) ) ;
#41767=CARTESIAN_POINT ( 'NONE',  ( -0.2700868329615992991, 1.134086821910841758, 0.1585113167840819515 ) ) ;
#41840=CARTESIAN_POINT ( 'NONE',  ( 0.2710477321170861043, 1.856769674693915295, 0.1570371412841552461 ) ) ;
#42346=CARTESIAN_POINT ( 'NONE',  ( 2.372150492836605294E-17, -1.268531780058464091E-17, 0.1937007874015748143 ) ) ;
#42454=DIRECTION ( 'NONE',  ( -0.000000000000000000, -1.000000000000000000, -0.000000000000000000 ) ) ;
#42667=CARTESIAN_POINT ( 'NONE',  ( 0.2223504907588284285, 1.906774035320677685, 0.2207610229706957194 ) ) ;
#42675=LINE ( 'NONE', #35963, #7675 ) ;
#42752=CARTESIAN_POINT ( 'NONE',  ( 0.1574803149606299746, 0.5905511811023621549, 0.000000000000000000 ) ) ;
#42753=( NAMED_UNIT ( * ) SI_UNIT ( $, .STERADIAN. ) SOLID_ANGLE_UNIT ( ) );
#42841=ORIENTED_EDGE ( 'NONE', *, *, #20396, .T. ) ;
#43147=CARTESIAN_POINT ( 'NONE',  ( -0.2908506741759562808, 1.813884536108223866, 0.1160749510518452737 ) ) ;
#43286=EDGE_CURVE ( 'NONE', #28541, #1243, #81014, .T. ) ;
#43652=CARTESIAN_POINT ( 'NONE',  ( 0.000000000000000000, 0.5905511811023621549, 0.000000000000000000 ) ) ;
#43771=DIMENSIONAL_EXPONENTS ( 1.000000000000000000, 0.000000000000000000, 0.000000000000000000, 0.000000000000000000, 0.000000000000000000, 0.000000000000000000, 0.000000000000000000 ) ;
#43794=CIRCLE ( 'NONE', #72082, 0.3129921259842521897 ) ;
#44030=ADVANCED_FACE ( 'NONE', ( #79851, #28893 ), #81086, .T. ) ;
#44138=CARTESIAN_POINT ( 'NONE',  ( 0.000000000000000000, 0.5905511811023621549, 0.000000000000000000 ) ) ;
#44200=DIRECTION ( 'NONE',  ( -0.000000000000000000, -1.000000000000000000, -0.000000000000000000 ) ) ;
#44356=SURFACE_STYLE_FILL_AREA ( #17085 ) ;
#44374=CARTESIAN_POINT ( 'NONE',  ( -0.01578888928619379128, 1.954428616053096146, 0.3129921259842520787 ) ) ;
#44637=B_SPLINE_CURVE_WITH_KNOTS ( 'NONE', 3,
 ( #969, #45544, #39241, #39667, #26623, #32511, #64088, #33362, #52694, #20733, #59435, #71242, #8107, #78819, #70827, #27449, #57755, #64925, #117, #7263, #21148, #65357, #46803, #59025, #72494, #33773, #27032, #46384 ),
 .UNSPECIFIED., .F., .F.,
 ( 4, 2, 2, 2, 2, 2, 2, 2, 2, 2, 2, 2, 2, 4 ),
 ( 0.06078874980787866283, 0.06175978776771125223, 0.06273082572754384856, 0.06370186368737643101, 0.06467290164720902734, 0.06564393960704162367, 0.06661497756687420613, 0.06855705348653938491, 0.06952809144637198124, 0.07049912940620456370, 0.07244120532586975636, 0.07341224328570235269, 0.07438328124553496290, 0.07632535716520016944 ),
 .UNSPECIFIED. ) ;
#44963=CIRCLE ( 'NONE', #69216, 0.1574803149606299746 ) ;
#44965=ORIENTED_EDGE ( 'NONE', *, *, #17897, .F. ) ;
#45544=CARTESIAN_POINT ( 'NONE',  ( 0.1455242698426520154, 1.053217739199509007, 0.2773898834120265833 ) ) ;
#45568=DIRECTION ( 'NONE',  ( -0.000000000000000000, -1.000000000000000000, -0.000000000000000000 ) ) ;
#45743=CARTESIAN_POINT ( 'NONE',  ( -0.01219799715822228459, 1.075705580628688374, 0.2362204724409448509 ) ) ;
#45776=CIRCLE ( 'NONE', #57847, 0.1937007874015747588 ) ;
#45830=LINE ( 'NONE', #71529, #41095 ) ;
#45853=AXIS2_PLACEMENT_3D ( 'NONE', #59018, #10589, #3026 ) ;
#46070=VECTOR ( 'NONE', #23327, 39.37007874015748854 ) ;
#46228=ORIENTED_EDGE ( 'NONE', *, *, #76419, .F. ) ;
#46243=ORIENTED_EDGE ( 'NONE', *, *, #14549, .F. ) ;
#46384=CARTESIAN_POINT ( 'NONE',  ( 0.3129921259842520787, 1.496062992125984259, 0.000000000000000000 ) ) ;
#46578=ORIENTED_EDGE ( 'NONE', *, *, #57708, .T. ) ;
#46803=CARTESIAN_POINT ( 'NONE',  ( 0.3125698167429954988, 1.368940321741649369, 0.01652806838128066322 ) ) ;
#46874=ORIENTED_EDGE ( 'NONE', *, *, #16485, .T. ) ;
#46924=CARTESIAN_POINT ( 'NONE',  ( -2.199130528046420221E-22, 1.075705580628688596, 0.2362204724409449064 ) ) ;
#46995=CARTESIAN_POINT ( 'NONE',  ( -0.1248512358867407135, 1.054133277639911714, 0.2754420493137687553 ) ) ;
#47253=CARTESIAN_POINT ( 'NONE',  ( -0.2321974025225331806, 1.091524521067366083, 0.2110349409267623655 ) ) ;
#47295=CARTESIAN_POINT ( 'NONE',  ( 0.000000000000000000, 0.7086614173228346081, 0.000000000000000000 ) ) ;
#47320=CARTESIAN_POINT ( 'NONE',  ( 0.01582383426708340937, 1.954428616053095924, 0.3129921259842521342 ) ) ;
#47545=DIRECTION ( 'NONE',  ( 0.000000000000000000, 1.000000000000000000, 0.000000000000000000 ) ) ;
#47809=CARTESIAN_POINT ( 'NONE',  ( 0.000000000000000000, 0.000000000000000000, -0.1937007874015747588 ) ) ;
#48090=ORIENTED_EDGE ( 'NONE', *, *, #79779, .T. ) ;
#48158=CARTESIAN_POINT ( 'NONE',  ( 0.3120460330268322036, 1.650912851539013682, 0.02472967731811865147 ) ) ;
#48733=ORIENTED_EDGE ( 'NONE', *, *, #19980, .T. ) ;
#49008=VERTEX_POINT ( 'NONE', #16560 ) ;
#49189=EDGE_CURVE ( 'NONE', #25849, #21435, #59593, .T. ) ;
#49398=CYLINDRICAL_SURFACE ( 'NONE', #25004, 0.3129921259842520787 ) ;
#49806=FACE_OUTER_BOUND ( 'NONE', #9096, .T. ) ;
#50039=ORIENTED_EDGE ( 'NONE', *, *, #83256, .T. ) ;
#50111=LINE ( 'NONE', #25, #68810 ) ;
#50650=AXIS2_PLACEMENT_3D ( 'NONE', #72514, #45568, #27056 ) ;
#50736=EDGE_CURVE ( 'NONE', #7519, #1243, #35515, .T. ) ;
#51517=DIRECTION ( 'NONE',  ( -0.000000000000000000, -1.000000000000000000, -0.000000000000000000 ) ) ;
#51725=CARTESIAN_POINT ( 'NONE',  ( 0.04852021190738116385, 1.072605569307989226, 0.2413719949950524080 ) ) ;
#51918=AXIS2_PLACEMENT_3D ( 'NONE', #80166, #41423, #21647 ) ;
#52043=DIRECTION ( 'NONE',  ( 0.000000000000000000, 0.000000000000000000, -1.000000000000000000 ) ) ;
#52104=EDGE_CURVE ( 'NONE', #15218, #14378, #54564, .T. ) ;
#52458=CYLINDRICAL_SURFACE ( 'NONE', #75188, 0.2165354330708661457 ) ;
#52523=ORIENTED_EDGE ( 'NONE', *, *, #78534, .F. ) ;
#52563=CARTESIAN_POINT ( 'NONE',  ( 0.06049490571020648549, 1.070753598490859382, 0.2444952571283235676 ) ) ;
#52694=CARTESIAN_POINT ( 'NONE',  ( 0.2390676544208471532, 1.098169981481509350, 0.2023185670810682124 ) ) ;
#52958=VECTOR ( 'NONE', #14607, 39.37007874015748143 ) ;
#52967=EDGE_LOOP ( 'NONE', ( #63219, #1213 ) ) ;
#53024=EDGE_CURVE ( 'NONE', #8617, #1453, #14020, .T. ) ;
#53371=CIRCLE ( 'NONE', #6325, 0.3129921259842520787 ) ;
#53659=EDGE_CURVE ( 'NONE', #15414, #1453, #76976, .T. ) ;
#53721=CARTESIAN_POINT ( 'NONE',  ( -0.1341536278048670039, 1.050682278017461835, 0.2827841492639485144 ) ) ;
#53976=DIRECTION ( 'NONE',  ( 0.000000000000000000, 0.000000000000000000, -1.000000000000000000 ) ) ;
#54046=CARTESIAN_POINT ( 'NONE',  ( 0.2768633925643534388, 1.846642183492231748, 0.1464305347622791575 ) ) ;
#54136=DIRECTION ( 'NONE',  ( 0.000000000000000000, -0.000000000000000000, 1.000000000000000000 ) ) ;
#54170=CIRCLE ( 'NONE', #12546, 0.2736220472440938911 ) ;
#54214=EDGE_LOOP ( 'NONE', ( #5671, #6197, #67699 ) ) ;
#54459=DIRECTION ( 'NONE',  ( -0.000000000000000000, -1.000000000000000000, -0.000000000000000000 ) ) ;
#54467=CARTESIAN_POINT ( 'NONE',  ( 0.2492559019816136257, 1.884140522857724376, 0.1894193705508290526 ) ) ;
#54564=B_SPLINE_CURVE_WITH_KNOTS ( 'NONE', 3,
 ( #32971, #7733, #13216, #33400, #1417, #78443, #27907, #14472, #38862, #58639, #1007, #40126, #8145, #72942, #41767, #29148, #36288, #47253, #66635, #74193, #35884, #61130, #74611, #28319 ),
 .UNSPECIFIED., .F., .F.,
 ( 4, 2, 2, 2, 2, 2, 2, 2, 2, 2, 2, 4 ),
 ( 0.03819530504429712037, 0.04014388769883309172, 0.04209247035336907000, 0.04404105300790504135, 0.04598963566244101964, 0.04696392698970900531, 0.04793821831697699098, 0.04891250964424497666, 0.04988680097151296233, 0.05183538362604894062, 0.05280967495331692629, 0.05378396628058491891 ),
 .UNSPECIFIED. ) ;
#54633=AXIS2_PLACEMENT_3D ( 'NONE', #67940, #54459, #80586 ) ;
#54688=DIRECTION ( 'NONE',  ( 0.000000000000000000, 0.000000000000000000, 1.000000000000000000 ) ) ;
#55224=ORIENTED_EDGE ( 'NONE', *, *, #35564, .F. ) ;
#55620=ADVANCED_FACE ( 'NONE', ( #32895 ), #72458, .F. ) ;
#55780=CARTESIAN_POINT ( 'NONE',  ( -0.3005583989984065840, 1.777033769787525808, 0.08778744816744185608 ) ) ;
#55908=CARTESIAN_POINT ( 'NONE',  ( 0.000000000000000000, 0.7086614173228346081, -0.3129921259842521897 ) ) ;
#56200=CARTESIAN_POINT ( 'NONE',  ( -0.1502557399355928802, 1.937763785080233836, 0.2750001312974072465 ) ) ;
#56554=CONICAL_SURFACE ( 'NONE', #40482, 0.3129921259842520787, 0.7853981633974533860 ) ;
#56606=CARTESIAN_POINT ( 'NONE',  ( -0.2003255369053823787, 1.919404900195578856, 0.2409235081687154112 ) ) ;
#56710=DIRECTION ( 'NONE',  ( 0.000000000000000000, -1.000000000000000000, -0.000000000000000000 ) ) ;
#56734=DIRECTION ( 'NONE',  ( 0.000000000000000000, 0.000000000000000000, 1.000000000000000000 ) ) ;
#56783=FACE_OUTER_BOUND ( 'NONE', #383, .T. ) ;
#56918=EDGE_CURVE ( 'NONE', #7519, #16433, #6925, .T. ) ;
#56939=DIRECTION ( 'NONE',  ( 0.000000000000000000, 0.000000000000000000, -1.000000000000000000 ) ) ;
#57013=CARTESIAN_POINT ( 'NONE',  ( -0.2316604258778182934, 1.900147917493397953, 0.2109207562938686387 ) ) ;
#57254=AXIS2_PLACEMENT_3D ( 'NONE', #67650, #34834, #16312 ) ;
#57287=CARTESIAN_POINT ( 'NONE',  ( 0.000000000000000000, -1.268531780058464091E-17, -0.1937007874015748143 ) ) ;
#57386=AXIS2_PLACEMENT_3D ( 'NONE', #24317, #56710, #68536 ) ;
#57429=CARTESIAN_POINT ( 'NONE',  ( -0.2766439779403090937, 1.847060205936300159, 0.1468512772251157894 ) ) ;
#57619=ORIENTED_EDGE ( 'NONE', *, *, #8988, .F. ) ;
#57708=EDGE_CURVE ( 'NONE', #15414, #75751, #44963, .T. ) ;
#57755=CARTESIAN_POINT ( 'NONE',  ( 0.3030237754406461814, 1.228860182587816929, 0.07866021050574804885 ) ) ;
#57847=AXIS2_PLACEMENT_3D ( 'NONE', #43652, #63035, #18429 ) ;
#58306=ORIENTED_EDGE ( 'NONE', *, *, #33733, .F. ) ;
#58335=VERTEX_POINT ( 'NONE', #2374 ) ;
#58362=CARTESIAN_POINT ( 'NONE',  ( 0.000000000000000000, 2.185078740157480937, 0.4527559055118110520 ) ) ;
#58639=CARTESIAN_POINT ( 'NONE',  ( -0.2965319783527583519, 1.197814162742229627, 0.1004664927356394566 ) ) ;
#58856=ORIENTED_EDGE ( 'NONE', *, *, #73238, .F. ) ;
#59000=MANIFOLD_SOLID_BREP ( 'Chamfer1', #72927 ) ;
#59018=CARTESIAN_POINT ( 'NONE',  ( 0.000000000000000000, 0.7086614173228346081, 0.4527559055118110520 ) ) ;
#59025=CARTESIAN_POINT ( 'NONE',  ( 0.3128291612561666657, 1.393967258436938472, 0.01053485884714776798 ) ) ;
#59217=ADVANCED_FACE ( 'NONE', ( #63324 ), #26693, .T. ) ;
#59435=CARTESIAN_POINT ( 'NONE',  ( 0.2588821398346105584, 1.118542505099386908, 0.1762126857782035649 ) ) ;
#59593=CIRCLE ( 'NONE', #67736, 0.1937007874015747588 ) ;
#60011=AXIS2_PLACEMENT_3D ( 'NONE', #65133, #7469, #32293 ) ;
#60012=EDGE_LOOP ( 'NONE', ( #7227, #72780 ) ) ;
#60787=CARTESIAN_POINT ( 'NONE',  ( 0.3129921259842520787, 1.496062992125984259, 0.000000000000000000 ) ) ;
#60807=PRODUCT_DEFINITION_SHAPE ( 'NONE', 'NONE',  #32108 ) ;
#60877=( NAMED_UNIT ( * ) PLANE_ANGLE_UNIT ( ) SI_UNIT ( $, .RADIAN. ) );
#60952=ORIENTED_EDGE ( 'NONE', *, *, #50736, .T. ) ;
#61130=CARTESIAN_POINT ( 'NONE',  ( -0.1565620680560287081, 1.056197359954963222, 0.2713048536997808569 ) ) ;
#61199=CARTESIAN_POINT ( 'NONE',  ( 0.2607642859107343059, 1.870951849707525927, 0.1732250691923664654 ) ) ;
#61306=PRODUCT_DEFINITION_CONTEXT ( 'detailed design', #67026, 'design' ) ;
#61313=VECTOR ( 'NONE', #33784, 39.37007874015748143 ) ;
#61550=FACE_BOUND ( 'NONE', #15385, .T. ) ;
#61604=APPLICATION_CONTEXT ( 'automotive_design' ) ;
#61625=CARTESIAN_POINT ( 'NONE',  ( 0.3072681130597426091, 1.737353037853611948, 0.06208766824286577474 ) ) ;
#61876=DIRECTION ( 'NONE',  ( 0.000000000000000000, 0.000000000000000000, -1.000000000000000000 ) ) ;
#62017=AXIS2_PLACEMENT_3D ( 'NONE', #68744, #18636, #75483 ) ;
#62035=CARTESIAN_POINT ( 'NONE',  ( 0.1890927523439494273, 1.924543803844427581, 0.2498735643778251525 ) ) ;
#62110=CARTESIAN_POINT ( 'NONE',  ( -0.3095605055124933114, 1.709780007968088489, 0.04771746845409036847 ) ) ;
#62378=CARTESIAN_POINT ( 'NONE',  ( -0.3129921259842521897, 1.496062992125984259, 0.000000000000000000 ) ) ;
#62389=ADVANCED_FACE ( 'NONE', ( #56783 ), #75343, .T. ) ;
#62613=ORIENTED_EDGE ( 'NONE', *, *, #53024, .F. ) ;
#62659=CIRCLE ( 'NONE', #60011, 0.1937007874015748143 ) ;
#62936=DIRECTION ( 'NONE',  ( -0.000000000000000000, -1.000000000000000000, -0.000000000000000000 ) ) ;
#63035=DIRECTION ( 'NONE',  ( -0.000000000000000000, -1.000000000000000000, -0.000000000000000000 ) ) ;
#63045=CARTESIAN_POINT ( 'NONE',  ( 0.000000000000000000, 2.145669291338582418, 0.000000000000000000 ) ) ;
#63219=ORIENTED_EDGE ( 'NONE', *, *, #33733, .T. ) ;
#63324=FACE_OUTER_BOUND ( 'NONE', #66310, .T. ) ;
#63753=CARTESIAN_POINT ( 'NONE',  ( -0.2707102524865197535, 1.857296401297248600, 0.1576108120785336686 ) ) ;
#64088=CARTESIAN_POINT ( 'NONE',  ( 0.2151207158954171472, 1.080925587658431608, 0.2276473237265549121 ) ) ;
#64374=DIRECTION ( 'NONE',  ( 0.000000000000000000, 1.000000000000000000, 0.000000000000000000 ) ) ;
#64400=CARTESIAN_POINT ( 'NONE',  ( 0.000000000000000000, 0.7086614173228346081, -0.1574803149606299746 ) ) ;
#64521=ADVANCED_BREP_SHAPE_REPRESENTATION ( '', ( #59000, #22098 ), #75874 ) ;
#64581=ORIENTED_EDGE ( 'NONE', *, *, #50736, .F. ) ;
#64893=AXIS2_PLACEMENT_3D ( 'NONE', #42752, #68036, #54136 ) ;
#64925=CARTESIAN_POINT ( 'NONE',  ( 0.3061702621670817082, 1.250678700630301510, 0.06534988725049302449 ) ) ;
#64935=LINE ( 'NONE', #65786, #61313 ) ;
#65133=CARTESIAN_POINT ( 'NONE',  ( 0.000000000000000000, -1.268531780058464091E-17, 0.000000000000000000 ) ) ;
#65318=CARTESIAN_POINT ( 'NONE',  ( -0.3129921259842521897, 1.496062992125984259, 0.4921259842519685179 ) ) ;
#65322=EDGE_LOOP ( 'NONE', ( #69685, #36127, #18007, #57619 ) ) ;
#65357=CARTESIAN_POINT ( 'NONE',  ( 0.3123753919909370014, 1.356452634660756384, 0.02004157963777108628 ) ) ;
#65474=EDGE_CURVE ( 'NONE', #49008, #16433, #11869, .T. ) ;
#65786=CARTESIAN_POINT ( 'NONE',  ( 3.833048052449394218E-17, 0.000000000000000000, 0.3129921259842520787 ) ) ;
#66041=ORIENTED_EDGE ( 'NONE', *, *, #20353, .T. ) ;
#66053=FACE_OUTER_BOUND ( 'NONE', #30555, .T. ) ;
#66058=CIRCLE ( 'NONE', #24339, 0.2165354330708661457 ) ;
#66129=ORIENTED_EDGE ( 'NONE', *, *, #52104, .F. ) ;
#66310=EDGE_LOOP ( 'NONE', ( #52523, #26140, #20680, #62613 ) ) ;
#66409=DIRECTION ( 'NONE',  ( 0.000000000000000000, 0.000000000000000000, -1.000000000000000000 ) ) ;
#66635=CARTESIAN_POINT ( 'NONE',  ( -0.2160876265729054779, 1.080600139074564536, 0.2277452782751286098 ) ) ;
#66833=DIRECTION ( 'NONE',  ( -0.000000000000000000, -1.000000000000000000, -0.000000000000000000 ) ) ;
#67026=APPLICATION_CONTEXT ( 'automotive_design' ) ;
#67404=CIRCLE ( 'NONE', #45853, 0.2165354330708661457 ) ;
#67530=CARTESIAN_POINT ( 'NONE',  ( 0.1641164824122239851, 1.933755502706929530, 0.2669431538071869725 ) ) ;
#67650=CARTESIAN_POINT ( 'NONE',  ( 0.000000000000000000, 0.000000000000000000, 0.000000000000000000 ) ) ;
#67699=ORIENTED_EDGE ( 'NONE', *, *, #35564, .T. ) ;
#67716=ORIENTED_EDGE ( 'NONE', *, *, #16485, .F. ) ;
#67736=AXIS2_PLACEMENT_3D ( 'NONE', #82994, #77096, #76677 ) ;
#67940=CARTESIAN_POINT ( 'NONE',  ( 0.000000000000000000, 2.185078740157480937, 0.4527559055118110520 ) ) ;
#68036=DIRECTION ( 'NONE',  ( 0.000000000000000000, 1.000000000000000000, 0.000000000000000000 ) ) ;
#68041=CARTESIAN_POINT ( 'NONE',  ( 3.833048050305355326E-17, 1.954428616053095924, 0.3129921259842520787 ) ) ;
#68178=MECHANICAL_DESIGN_GEOMETRIC_PRESENTATION_REPRESENTATION('',(#2325),#33200);
#68335=ORIENTED_EDGE ( 'NONE', *, *, #56918, .F. ) ;
#68437=CARTESIAN_POINT ( 'NONE',  ( -0.2977726995931780918, 1.789762378577807400, 0.09694807015762342550 ) ) ;
#68536=DIRECTION ( 'NONE',  ( 0.000000000000000000, 0.000000000000000000, -1.000000000000000000 ) ) ;
#68690=CARTESIAN_POINT ( 'NONE',  ( 0.3129921259842521897, 0.7086614173228346081, 0.000000000000000000 ) ) ;
#68744=CARTESIAN_POINT ( 'NONE',  ( 0.000000000000000000, 2.185039370078740273, 0.000000000000000000 ) ) ;
#68810=VECTOR ( 'NONE', #44200, 39.37007874015748143 ) ;
#68835=EDGE_LOOP ( 'NONE', ( #44965, #50039, #7885, #34267 ) ) ;
#68838=CARTESIAN_POINT ( 'NONE',  ( 0.000000000000000000, 0.000000000000000000, 0.000000000000000000 ) ) ;
#68902=EDGE_CURVE ( 'NONE', #15218, #58335, #36704, .T. ) ;
#68976=B_SPLINE_CURVE_WITH_KNOTS ( 'NONE', 3,
 ( #60787, #34716, #9868, #81000, #3140, #48158, #80180, #22901, #61625, #74682, #21660, #3967, #35537, #54046, #41840, #61199, #28803, #54467, #23314, #17028, #42667, #16609, #62035, #67530, #41436, #22077, #29630, #3556, #74266, #79760, #47320, #2725 ),
 .UNSPECIFIED., .F., .F.,
 ( 4, 2, 2, 2, 2, 2, 2, 2, 2, 2, 2, 2, 2, 2, 2, 4 ),
 ( 3.680777123389603761E-21, 0.002389845404268378572, 0.003584768106402557667, 0.004779690808536737195, 0.007169536212805114467, 0.008364458914939303102, 0.009559381617073493473, 0.01075430431920768211, 0.01135176567027477643, 0.01194922702134187248, 0.01314414972347606979, 0.01433907242561027057, 0.01553399512774447135, 0.01672891782987866865, 0.01792384053201287117, 0.01911876323414707021 ),
 .UNSPECIFIED. ) ;
#69081=AXIS2_PLACEMENT_3D ( 'NONE', #68838, #62936, #10364 ) ;
#69199=CARTESIAN_POINT ( 'NONE',  ( 1.928577636452524918E-17, 0.7086614173228346081, 0.1574803149606299746 ) ) ;
#69216=AXIS2_PLACEMENT_3D ( 'NONE', #47295, #72572, #35512 ) ;
#69331=VERTEX_POINT ( 'NONE', #57287 ) ;
#69669=CARTESIAN_POINT ( 'NONE',  ( -0.03146197511274030634, 1.953969648464710884, 0.3118041613806297740 ) ) ;
#69685=ORIENTED_EDGE ( 'NONE', *, *, #30068, .F. ) ;
#70690=LINE ( 'NONE', #38696, #78725 ) ;
#70827=CARTESIAN_POINT ( 'NONE',  ( 0.2941356937468260768, 1.187227223647445484, 0.1081275479939705769 ) ) ;
#71137=CARTESIAN_POINT ( 'NONE',  ( -0.3129921259842520787, 1.496062992125984259, 2.300774849103979725E-17 ) ) ;
#71242=CARTESIAN_POINT ( 'NONE',  ( 0.2699421371814171300, 1.133868921557234843, 0.1587517418123144675 ) ) ;
#71316=ORIENTED_EDGE ( 'NONE', *, *, #83256, .F. ) ;
#71382=ADVANCED_FACE ( 'NONE', ( #81111 ), #3671, .T. ) ;
#71434=ORIENTED_EDGE ( 'NONE', *, *, #78534, .T. ) ;
#71458=UNCERTAINTY_MEASURE_WITH_UNIT (LENGTH_MEASURE( 1.000000000000000082E-05 ), #23816, 'distance_accuracy_value', 'NONE');
#71529=CARTESIAN_POINT ( 'NONE',  ( 0.000000000000000000, 2.145669291338582418, -0.3129921259842520787 ) ) ;
#72082=AXIS2_PLACEMENT_3D ( 'NONE', #78082, #79752, #20828 ) ;
#72458=CYLINDRICAL_SURFACE ( 'NONE', #5999, 0.4921259842519685179 ) ;
#72494=CARTESIAN_POINT ( 'NONE',  ( 0.3128952852777661664, 1.406554901604258889, 0.008038607527843355527 ) ) ;
#72514=CARTESIAN_POINT ( 'NONE',  ( 0.000000000000000000, 0.7086614173228346081, 0.000000000000000000 ) ) ;
#72572=DIRECTION ( 'NONE',  ( -0.000000000000000000, -1.000000000000000000, -0.000000000000000000 ) ) ;
#72688=CARTESIAN_POINT ( 'NONE',  ( -0.1150178391344491569, 1.057423598266512332, 0.2689098498627903733 ) ) ;
#72780=ORIENTED_EDGE ( 'NONE', *, *, #53024, .T. ) ;
#72906=CARTESIAN_POINT ( 'NONE',  ( 0.000000000000000000, 2.185039370078740273, 0.000000000000000000 ) ) ;
#72927=CLOSED_SHELL ( 'NONE', ( #11014, #1297, #55620, #27002, #62389, #71382, #14869, #36321, #6346, #59217, #44030, #80245, #40409, #10309, #12372, #7943 ) ) ;
#72942=CARTESIAN_POINT ( 'NONE',  ( -0.2749671762622359350, 1.142275244175160909, 0.1498262158730659654 ) ) ;
#73132=AXIS2_PLACEMENT_3D ( 'NONE', #63045, #81181, #35720 ) ;
#73166=ORIENTED_EDGE ( 'NONE', *, *, #25084, .T. ) ;
#73238=EDGE_CURVE ( 'NONE', #81942, #69331, #8939, .T. ) ;
#73490=AXIS2_PLACEMENT_3D ( 'NONE', #20602, #77850, #40780 ) ;
#73542=CYLINDRICAL_SURFACE ( 'NONE', #26401, 0.4921259842519685179 ) ;
#74193=CARTESIAN_POINT ( 'NONE',  ( -0.1875998866324375958, 1.067055059779716597, 0.2508381535278075281 ) ) ;
#74266=CARTESIAN_POINT ( 'NONE',  ( 0.06306398308594768354, 1.952040271819099004, 0.3069791477017838055 ) ) ;
#74485=CARTESIAN_POINT ( 'NONE',  ( 0.000000000000000000, 2.185039370078740273, 0.000000000000000000 ) ) ;
#74611=CARTESIAN_POINT ( 'NONE',  ( -0.1455973158445646731, 1.053234027224559943, 0.2773552301749948046 ) ) ;
#74682=CARTESIAN_POINT ( 'NONE',  ( 0.3006637500733741475, 1.776489521407567551, 0.08741570540071638695 ) ) ;
#74737=FILL_AREA_STYLE_COLOUR ( '', #21132 ) ;
#74758=CARTESIAN_POINT ( 'NONE',  ( -0.07815110806776767727, 1.950626090833269766, 0.3034832608173697599 ) ) ;
#74851=AXIS2_PLACEMENT_3D ( 'NONE', #15486, #66833, #66409 ) ;
#75063=VERTEX_POINT ( 'NONE', #46924 ) ;
#75188=AXIS2_PLACEMENT_3D ( 'NONE', #58362, #25958, #40269 ) ;
#75343=CYLINDRICAL_SURFACE ( 'NONE', #19797, 0.1574803149606299746 ) ;
#75483=DIRECTION ( 'NONE',  ( 0.000000000000000000, 0.000000000000000000, 1.000000000000000000 ) ) ;
#75521=CARTESIAN_POINT ( 'NONE',  ( 3.833048052449394218E-17, 2.145669291338582418, 0.3129921259842520787 ) ) ;
#75583=CARTESIAN_POINT ( 'NONE',  ( -0.3129921259842521342, 1.527825669364019756, 5.602422643256820041E-18 ) ) ;
#75599=ORIENTED_EDGE ( 'NONE', *, *, #36496, .T. ) ;
#75751=VERTEX_POINT ( 'NONE', #69199 ) ;
#75874=( GEOMETRIC_REPRESENTATION_CONTEXT ( 3 ) GLOBAL_UNCERTAINTY_ASSIGNED_CONTEXT ( ( #71458 ) ) GLOBAL_UNIT_ASSIGNED_CONTEXT ( ( #23816, #60877, #42753 ) ) REPRESENTATION_CONTEXT ( 'NONE', 'WORKASPACE' ) );
#76091=ORIENTED_EDGE ( 'NONE', *, *, #17897, .T. ) ;
#76103=CONICAL_SURFACE ( 'NONE', #881, 0.3129921259842520787, 0.7853981633974533860 ) ;
#76132=SHAPE_REPRESENTATION ( 'Spindle Dowel Pin', ( #22098 ), #75874 ) ;
#76162=ORIENTED_EDGE ( 'NONE', *, *, #28583, .F. ) ;
#76419=EDGE_CURVE ( 'NONE', #28541, #31638, #54170, .T. ) ;
#76473=ORIENTED_EDGE ( 'NONE', *, *, #65474, .F. ) ;
#76558=CARTESIAN_POINT ( 'NONE',  ( 0.000000000000000000, 0.7086614173228346081, 0.4527559055118110520 ) ) ;
#76677=DIRECTION ( 'NONE',  ( 0.000000000000000000, 0.000000000000000000, -1.000000000000000000 ) ) ;
#76976=LINE ( 'NONE', #38247, #38252 ) ;
#77096=DIRECTION ( 'NONE',  ( -0.000000000000000000, -1.000000000000000000, -0.000000000000000000 ) ) ;
#77427=CARTESIAN_POINT ( 'NONE',  ( 0.08317790770047603366, 1.066208230691911174, 0.2524721893675162532 ) ) ;
#77547=AXIS2_PLACEMENT_3D ( 'NONE', #7767, #40993, #20385 ) ;
#77639=ORIENTED_EDGE ( 'NONE', *, *, #28151, .F. ) ;
#77850=DIRECTION ( 'NONE',  ( -0.000000000000000000, -1.000000000000000000, -0.000000000000000000 ) ) ;
#78082=CARTESIAN_POINT ( 'NONE',  ( 0.000000000000000000, 0.7086614173228346081, 0.000000000000000000 ) ) ;
#78181=CARTESIAN_POINT ( 'NONE',  ( -2.199130528046420221E-22, 1.075705580628688596, 0.2362204724409449064 ) ) ;
#78443=CARTESIAN_POINT ( 'NONE',  ( -0.3114559808008819930, 1.319608357126878184, 0.03199222220977063907 ) ) ;
#78486=CARTESIAN_POINT ( 'NONE',  ( 0.000000000000000000, 0.000000000000000000, -0.3129921259842520787 ) ) ;
#78534=EDGE_CURVE ( 'NONE', #75751, #8617, #81529, .T. ) ;
#78693=CARTESIAN_POINT ( 'NONE',  ( 0.1148797229700118799, 1.057468328962668069, 0.2688218391471720037 ) ) ;
#78725=VECTOR ( 'NONE', #64374, 39.37007874015748143 ) ;
#78819=CARTESIAN_POINT ( 'NONE',  ( 0.2878949040089971434, 1.168214014193575956, 0.1242954387040235420 ) ) ;
#79100=EDGE_LOOP ( 'NONE', ( #46228, #33330, #64581, #19735 ) ) ;
#79365=ORIENTED_EDGE ( 'NONE', *, *, #68902, .F. ) ;
#79656=DIRECTION ( 'NONE',  ( 0.000000000000000000, -0.000000000000000000, 1.000000000000000000 ) ) ;
#79752=DIRECTION ( 'NONE',  ( -0.000000000000000000, -1.000000000000000000, -0.000000000000000000 ) ) ;
#79760=CARTESIAN_POINT ( 'NONE',  ( 0.03185741929354787838, 1.953955006892923674, 0.3117665279056321959 ) ) ;
#79779=EDGE_CURVE ( 'NONE', #21435, #69331, #3625, .T. ) ;
#79851=FACE_BOUND ( 'NONE', #60012, .T. ) ;
#79987=ORIENTED_EDGE ( 'NONE', *, *, #43286, .F. ) ;
#80166=CARTESIAN_POINT ( 'NONE',  ( 0.000000000000000000, 0.7086614173228346081, 0.000000000000000000 ) ) ;
#80173=CYLINDRICAL_SURFACE ( 'NONE', #54633, 0.2165354330708661457 ) ;
#80180=CARTESIAN_POINT ( 'NONE',  ( 0.3116086372737535415, 1.665959576555773314, 0.02998912175037303507 ) ) ;
#80245=ADVANCED_FACE ( 'NONE', ( #23385 ), #37260, .T. ) ;
#80586=DIRECTION ( 'NONE',  ( 0.000000000000000000, 0.000000000000000000, -1.000000000000000000 ) ) ;
#80787=AXIS2_PLACEMENT_3D ( 'NONE', #13353, #32698, #52043 ) ;
#81000=CARTESIAN_POINT ( 'NONE',  ( 0.3127753386821575665, 1.605323575777892087, 0.01202575393854246610 ) ) ;
#81014=LINE ( 'NONE', #75521, #46070 ) ;
#81086=PLANE ( 'NONE',  #64893 ) ;
#81088=CARTESIAN_POINT ( 'NONE',  ( 2.372150492836604986E-17, 0.5905511811023621549, 0.1937007874015747588 ) ) ;
#81111=FACE_OUTER_BOUND ( 'NONE', #14207, .T. ) ;
#81181=DIRECTION ( 'NONE',  ( -0.000000000000000000, -1.000000000000000000, -0.000000000000000000 ) ) ;
#81335=PLANE ( 'NONE',  #9758 ) ;
#81468=( CONVERSION_BASED_UNIT ( 'INCH', #36831 ) LENGTH_UNIT ( ) NAMED_UNIT ( #24430 ) );
#81488=CARTESIAN_POINT ( 'NONE',  ( -0.3126874984954384762, 1.620889671569059942, 0.01505614298776670329 ) ) ;
#81529=LINE ( 'NONE', #23849, #35498 ) ;
#81901=CARTESIAN_POINT ( 'NONE',  ( -0.3122834589929986970, 1.651567687059297240, 0.02415997947403120821 ) ) ;
#81942=VERTEX_POINT ( 'NONE', #42346 ) ;
#82709=CARTESIAN_POINT ( 'NONE',  ( -0.1080761259423674570, 1.946643253402353224, 0.2941585223818156680 ) ) ;
#82994=CARTESIAN_POINT ( 'NONE',  ( 0.000000000000000000, 0.5905511811023621549, 0.000000000000000000 ) ) ;
#83256=EDGE_CURVE ( 'NONE', #75063, #14378, #34422, .T. ) ;
ENDSEC;
END-ISO-10303-21;
